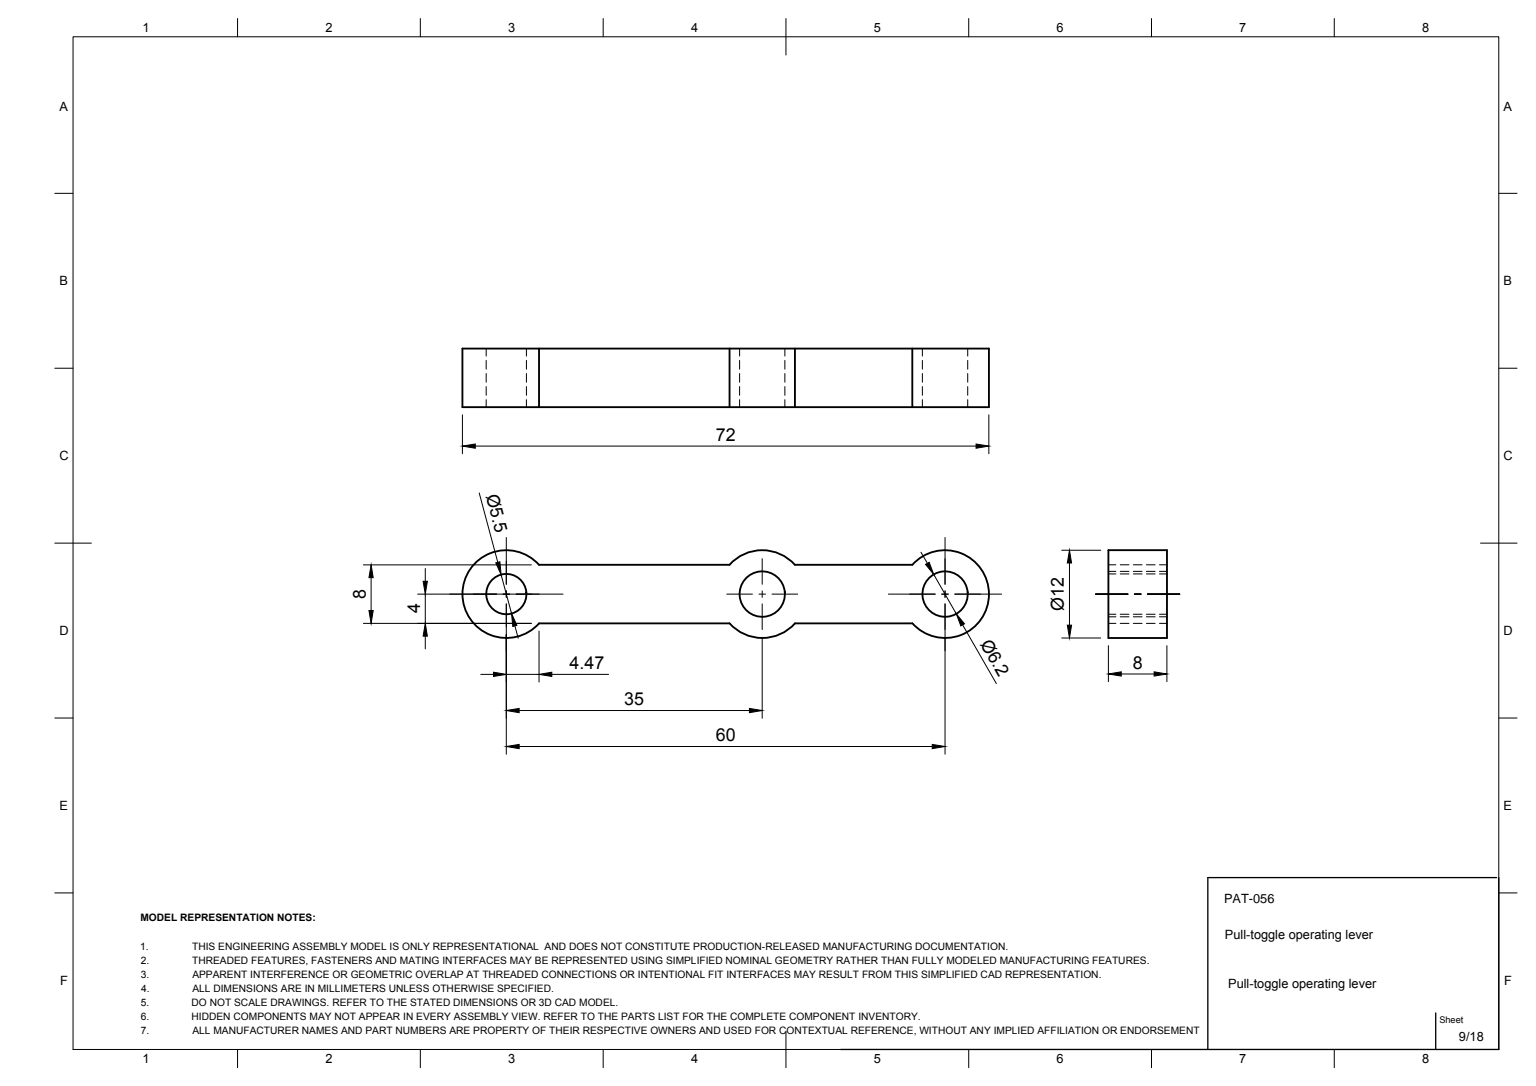
ISO-10303-21;
HEADER;
/* Generated by software containing ST-Developer
 * from STEP Tools, Inc. (www.steptools.com) 
 */

FILE_DESCRIPTION(
/* description */ ('Hook toggle clamp'),
/* implementation_level */ '2;1');

FILE_NAME(
/* name */ 'Pull-toggle operating lever.step',
/* time_stamp */ '2026-10-27T21:56:56-07:00',
/* author */ (''),
/* organization */ (''),
/* preprocessor_version */ 'ST-DEVELOPER v20.2',
/* originating_system */ 'Autodesk Translation Framework v15.17.0.0',
/* authorisation */ '');

FILE_SCHEMA (('AUTOMOTIVE_DESIGN { 1 0 10303 214 3 1 1 }'));
ENDSEC;

DATA;
#10=MECHANICAL_DESIGN_GEOMETRIC_PRESENTATION_REPRESENTATION('',(#192),#5458);
#158=SHAPE_REPRESENTATION_RELATIONSHIP('SRR','None',#5540,#175);
#175=ADVANCED_BREP_SHAPE_REPRESENTATION('',(#209),#5442);
#192=STYLED_ITEM('',(#5710),#209);
#209=MANIFOLD_SOLID_BREP('Body1',#2973);
#243=FACE_BOUND('',#653,.T.);
#244=FACE_BOUND('',#654,.T.);
#245=FACE_BOUND('',#655,.T.);
#246=FACE_BOUND('',#660,.T.);
#247=FACE_BOUND('',#661,.T.);
#248=FACE_BOUND('',#662,.T.);
#328=PLANE('',#3281);
#329=PLANE('',#3285);
#330=PLANE('',#3290);
#331=PLANE('',#3292);
#332=PLANE('',#3293);
#333=PLANE('',#3294);
#454=FACE_OUTER_BOUND('',#648,.T.);
#455=FACE_OUTER_BOUND('',#649,.T.);
#456=FACE_OUTER_BOUND('',#650,.T.);
#457=FACE_OUTER_BOUND('',#651,.T.);
#458=FACE_OUTER_BOUND('',#652,.T.);
#459=FACE_OUTER_BOUND('',#656,.T.);
#460=FACE_OUTER_BOUND('',#657,.T.);
#461=FACE_OUTER_BOUND('',#658,.T.);
#462=FACE_OUTER_BOUND('',#659,.T.);
#463=FACE_OUTER_BOUND('',#663,.T.);
#464=FACE_OUTER_BOUND('',#664,.T.);
#465=FACE_OUTER_BOUND('',#665,.T.);
#466=FACE_OUTER_BOUND('',#666,.T.);
#648=EDGE_LOOP('',(#2299,#2300,#2301,#2302));
#649=EDGE_LOOP('',(#2303,#2304,#2305,#2306));
#650=EDGE_LOOP('',(#2307,#2308,#2309,#2310));
#651=EDGE_LOOP('',(#2311,#2312,#2313,#2314));
#652=EDGE_LOOP('',(#2315,#2316,#2317,#2318,#2319,#2320,#2321,#2322));
#653=EDGE_LOOP('',(#2323));
#654=EDGE_LOOP('',(#2324));
#655=EDGE_LOOP('',(#2325));
#656=EDGE_LOOP('',(#2326,#2327,#2328,#2329));
#657=EDGE_LOOP('',(#2330,#2331,#2332,#2333));
#658=EDGE_LOOP('',(#2334,#2335,#2336,#2337));
#659=EDGE_LOOP('',(#2338,#2339,#2340,#2341,#2342,#2343,#2344,#2345));
#660=EDGE_LOOP('',(#2346));
#661=EDGE_LOOP('',(#2347));
#662=EDGE_LOOP('',(#2348));
#663=EDGE_LOOP('',(#2349,#2350,#2351,#2352));
#664=EDGE_LOOP('',(#2353,#2354,#2355,#2356));
#665=EDGE_LOOP('',(#2357,#2358,#2359,#2360));
#666=EDGE_LOOP('',(#2361,#2362,#2363,#2364));
#913=LINE('',#4750,#1150);
#914=LINE('',#4756,#1151);
#915=LINE('',#4762,#1152);
#916=LINE('',#4767,#1153);
#917=LINE('',#4771,#1154);
#918=LINE('',#4775,#1155);
#919=LINE('',#4779,#1156);
#920=LINE('',#4783,#1157);
#921=LINE('',#4786,#1158);
#922=LINE('',#4789,#1159);
#923=LINE('',#4790,#1160);
#924=LINE('',#4794,#1161);
#925=LINE('',#4797,#1162);
#926=LINE('',#4799,#1163);
#927=LINE('',#4802,#1164);
#928=LINE('',#4804,#1165);
#929=LINE('',#4807,#1166);
#930=LINE('',#4809,#1167);
#931=LINE('',#4811,#1168);
#1150=VECTOR('',#3819,0.275);
#1151=VECTOR('',#3826,0.31);
#1152=VECTOR('',#3833,0.31);
#1153=VECTOR('',#3838,1.);
#1154=VECTOR('',#3841,1.);
#1155=VECTOR('',#3846,1.);
#1156=VECTOR('',#3849,1.);
#1157=VECTOR('',#3852,1.);
#1158=VECTOR('',#3855,1.);
#1159=VECTOR('',#3858,1.);
#1160=VECTOR('',#3859,1.);
#1161=VECTOR('',#3864,1.);
#1162=VECTOR('',#3867,1.);
#1163=VECTOR('',#3868,1.);
#1164=VECTOR('',#3873,1.);
#1165=VECTOR('',#3874,1.);
#1166=VECTOR('',#3877,1.);
#1167=VECTOR('',#3880,1.);
#1168=VECTOR('',#3883,1.);
#1294=CIRCLE('',#3270,0.275);
#1295=CIRCLE('',#3271,0.275);
#1296=CIRCLE('',#3273,0.31);
#1297=CIRCLE('',#3274,0.31);
#1298=CIRCLE('',#3276,0.31);
#1299=CIRCLE('',#3277,0.31);
#1300=CIRCLE('',#3279,0.6);
#1301=CIRCLE('',#3280,0.6);
#1302=CIRCLE('',#3282,0.6);
#1303=CIRCLE('',#3283,0.6);
#1304=CIRCLE('',#3284,0.6);
#1305=CIRCLE('',#3287,0.6);
#1306=CIRCLE('',#3289,0.6);
#1307=CIRCLE('',#3291,0.6);
#1481=VERTEX_POINT('',#4747);
#1482=VERTEX_POINT('',#4749);
#1483=VERTEX_POINT('',#4753);
#1484=VERTEX_POINT('',#4755);
#1485=VERTEX_POINT('',#4759);
#1486=VERTEX_POINT('',#4761);
#1487=VERTEX_POINT('',#4765);
#1488=VERTEX_POINT('',#4766);
#1489=VERTEX_POINT('',#4768);
#1490=VERTEX_POINT('',#4770);
#1491=VERTEX_POINT('',#4774);
#1492=VERTEX_POINT('',#4776);
#1493=VERTEX_POINT('',#4778);
#1494=VERTEX_POINT('',#4780);
#1495=VERTEX_POINT('',#4782);
#1496=VERTEX_POINT('',#4784);
#1497=VERTEX_POINT('',#4788);
#1498=VERTEX_POINT('',#4792);
#1499=VERTEX_POINT('',#4796);
#1500=VERTEX_POINT('',#4798);
#1501=VERTEX_POINT('',#4803);
#1502=VERTEX_POINT('',#4805);
#1776=EDGE_CURVE('',#1481,#1481,#1294,.T.);
#1777=EDGE_CURVE('',#1481,#1482,#913,.T.);
#1778=EDGE_CURVE('',#1482,#1482,#1295,.T.);
#1779=EDGE_CURVE('',#1483,#1483,#1296,.T.);
#1780=EDGE_CURVE('',#1483,#1484,#914,.T.);
#1781=EDGE_CURVE('',#1484,#1484,#1297,.T.);
#1782=EDGE_CURVE('',#1485,#1485,#1298,.T.);
#1783=EDGE_CURVE('',#1485,#1486,#915,.T.);
#1784=EDGE_CURVE('',#1486,#1486,#1299,.T.);
#1785=EDGE_CURVE('',#1487,#1488,#916,.T.);
#1786=EDGE_CURVE('',#1489,#1487,#1300,.T.);
#1787=EDGE_CURVE('',#1490,#1489,#917,.T.);
#1788=EDGE_CURVE('',#1490,#1488,#1301,.T.);
#1789=EDGE_CURVE('',#1491,#1490,#918,.T.);
#1790=EDGE_CURVE('',#1492,#1491,#1302,.T.);
#1791=EDGE_CURVE('',#1493,#1492,#919,.T.);
#1792=EDGE_CURVE('',#1494,#1493,#1303,.T.);
#1793=EDGE_CURVE('',#1495,#1494,#920,.T.);
#1794=EDGE_CURVE('',#1496,#1495,#1304,.T.);
#1795=EDGE_CURVE('',#1488,#1496,#921,.T.);
#1796=EDGE_CURVE('',#1497,#1489,#922,.T.);
#1797=EDGE_CURVE('',#1497,#1491,#923,.T.);
#1798=EDGE_CURVE('',#1498,#1497,#1305,.T.);
#1799=EDGE_CURVE('',#1492,#1498,#924,.T.);
#1800=EDGE_CURVE('',#1496,#1499,#925,.T.);
#1801=EDGE_CURVE('',#1500,#1495,#926,.T.);
#1802=EDGE_CURVE('',#1499,#1500,#1306,.T.);
#1803=EDGE_CURVE('',#1487,#1499,#927,.T.);
#1804=EDGE_CURVE('',#1500,#1501,#928,.T.);
#1805=EDGE_CURVE('',#1501,#1502,#1307,.T.);
#1806=EDGE_CURVE('',#1502,#1498,#929,.T.);
#1807=EDGE_CURVE('',#1501,#1494,#930,.T.);
#1808=EDGE_CURVE('',#1493,#1502,#931,.T.);
#2299=ORIENTED_EDGE('',*,*,#1776,.F.);
#2300=ORIENTED_EDGE('',*,*,#1777,.T.);
#2301=ORIENTED_EDGE('',*,*,#1778,.F.);
#2302=ORIENTED_EDGE('',*,*,#1777,.F.);
#2303=ORIENTED_EDGE('',*,*,#1779,.F.);
#2304=ORIENTED_EDGE('',*,*,#1780,.T.);
#2305=ORIENTED_EDGE('',*,*,#1781,.F.);
#2306=ORIENTED_EDGE('',*,*,#1780,.F.);
#2307=ORIENTED_EDGE('',*,*,#1782,.F.);
#2308=ORIENTED_EDGE('',*,*,#1783,.T.);
#2309=ORIENTED_EDGE('',*,*,#1784,.F.);
#2310=ORIENTED_EDGE('',*,*,#1783,.F.);
#2311=ORIENTED_EDGE('',*,*,#1785,.F.);
#2312=ORIENTED_EDGE('',*,*,#1786,.F.);
#2313=ORIENTED_EDGE('',*,*,#1787,.F.);
#2314=ORIENTED_EDGE('',*,*,#1788,.T.);
#2315=ORIENTED_EDGE('',*,*,#1788,.F.);
#2316=ORIENTED_EDGE('',*,*,#1789,.F.);
#2317=ORIENTED_EDGE('',*,*,#1790,.F.);
#2318=ORIENTED_EDGE('',*,*,#1791,.F.);
#2319=ORIENTED_EDGE('',*,*,#1792,.F.);
#2320=ORIENTED_EDGE('',*,*,#1793,.F.);
#2321=ORIENTED_EDGE('',*,*,#1794,.F.);
#2322=ORIENTED_EDGE('',*,*,#1795,.F.);
#2323=ORIENTED_EDGE('',*,*,#1776,.T.);
#2324=ORIENTED_EDGE('',*,*,#1779,.T.);
#2325=ORIENTED_EDGE('',*,*,#1782,.T.);
#2326=ORIENTED_EDGE('',*,*,#1787,.T.);
#2327=ORIENTED_EDGE('',*,*,#1796,.F.);
#2328=ORIENTED_EDGE('',*,*,#1797,.T.);
#2329=ORIENTED_EDGE('',*,*,#1789,.T.);
#2330=ORIENTED_EDGE('',*,*,#1797,.F.);
#2331=ORIENTED_EDGE('',*,*,#1798,.F.);
#2332=ORIENTED_EDGE('',*,*,#1799,.F.);
#2333=ORIENTED_EDGE('',*,*,#1790,.T.);
#2334=ORIENTED_EDGE('',*,*,#1800,.F.);
#2335=ORIENTED_EDGE('',*,*,#1794,.T.);
#2336=ORIENTED_EDGE('',*,*,#1801,.F.);
#2337=ORIENTED_EDGE('',*,*,#1802,.F.);
#2338=ORIENTED_EDGE('',*,*,#1803,.T.);
#2339=ORIENTED_EDGE('',*,*,#1802,.T.);
#2340=ORIENTED_EDGE('',*,*,#1804,.T.);
#2341=ORIENTED_EDGE('',*,*,#1805,.T.);
#2342=ORIENTED_EDGE('',*,*,#1806,.T.);
#2343=ORIENTED_EDGE('',*,*,#1798,.T.);
#2344=ORIENTED_EDGE('',*,*,#1796,.T.);
#2345=ORIENTED_EDGE('',*,*,#1786,.T.);
#2346=ORIENTED_EDGE('',*,*,#1778,.T.);
#2347=ORIENTED_EDGE('',*,*,#1781,.T.);
#2348=ORIENTED_EDGE('',*,*,#1784,.T.);
#2349=ORIENTED_EDGE('',*,*,#1801,.T.);
#2350=ORIENTED_EDGE('',*,*,#1793,.T.);
#2351=ORIENTED_EDGE('',*,*,#1807,.F.);
#2352=ORIENTED_EDGE('',*,*,#1804,.F.);
#2353=ORIENTED_EDGE('',*,*,#1799,.T.);
#2354=ORIENTED_EDGE('',*,*,#1806,.F.);
#2355=ORIENTED_EDGE('',*,*,#1808,.F.);
#2356=ORIENTED_EDGE('',*,*,#1791,.T.);
#2357=ORIENTED_EDGE('',*,*,#1785,.T.);
#2358=ORIENTED_EDGE('',*,*,#1795,.T.);
#2359=ORIENTED_EDGE('',*,*,#1800,.T.);
#2360=ORIENTED_EDGE('',*,*,#1803,.F.);
#2361=ORIENTED_EDGE('',*,*,#1807,.T.);
#2362=ORIENTED_EDGE('',*,*,#1792,.T.);
#2363=ORIENTED_EDGE('',*,*,#1808,.T.);
#2364=ORIENTED_EDGE('',*,*,#1805,.F.);
#2759=CYLINDRICAL_SURFACE('',#3269,0.275);
#2760=CYLINDRICAL_SURFACE('',#3272,0.31);
#2761=CYLINDRICAL_SURFACE('',#3275,0.31);
#2762=CYLINDRICAL_SURFACE('',#3278,0.6);
#2763=CYLINDRICAL_SURFACE('',#3286,0.6);
#2764=CYLINDRICAL_SURFACE('',#3288,0.6);
#2765=CYLINDRICAL_SURFACE('',#3295,0.6);
#2858=ADVANCED_FACE('',(#454),#2759,.F.);
#2859=ADVANCED_FACE('',(#455),#2760,.F.);
#2860=ADVANCED_FACE('',(#456),#2761,.F.);
#2861=ADVANCED_FACE('',(#457),#2762,.T.);
#2862=ADVANCED_FACE('',(#458,#243,#244,#245),#328,.F.);
#2863=ADVANCED_FACE('',(#459),#329,.T.);
#2864=ADVANCED_FACE('',(#460),#2763,.T.);
#2865=ADVANCED_FACE('',(#461),#2764,.T.);
#2866=ADVANCED_FACE('',(#462,#246,#247,#248),#330,.T.);
#2867=ADVANCED_FACE('',(#463),#331,.T.);
#2868=ADVANCED_FACE('',(#464),#332,.T.);
#2869=ADVANCED_FACE('',(#465),#333,.T.);
#2870=ADVANCED_FACE('',(#466),#2765,.T.);
#2973=CLOSED_SHELL('',(#2858,#2859,#2860,#2861,#2862,#2863,#2864,#2865,
#2866,#2867,#2868,#2869,#2870));
#3268=AXIS2_PLACEMENT_3D('',#4745,#3813,#3814);
#3269=AXIS2_PLACEMENT_3D('',#4746,#3815,#3816);
#3270=AXIS2_PLACEMENT_3D('',#4748,#3817,#3818);
#3271=AXIS2_PLACEMENT_3D('',#4751,#3820,#3821);
#3272=AXIS2_PLACEMENT_3D('',#4752,#3822,#3823);
#3273=AXIS2_PLACEMENT_3D('',#4754,#3824,#3825);
#3274=AXIS2_PLACEMENT_3D('',#4757,#3827,#3828);
#3275=AXIS2_PLACEMENT_3D('',#4758,#3829,#3830);
#3276=AXIS2_PLACEMENT_3D('',#4760,#3831,#3832);
#3277=AXIS2_PLACEMENT_3D('',#4763,#3834,#3835);
#3278=AXIS2_PLACEMENT_3D('',#4764,#3836,#3837);
#3279=AXIS2_PLACEMENT_3D('',#4769,#3839,#3840);
#3280=AXIS2_PLACEMENT_3D('',#4772,#3842,#3843);
#3281=AXIS2_PLACEMENT_3D('',#4773,#3844,#3845);
#3282=AXIS2_PLACEMENT_3D('',#4777,#3847,#3848);
#3283=AXIS2_PLACEMENT_3D('',#4781,#3850,#3851);
#3284=AXIS2_PLACEMENT_3D('',#4785,#3853,#3854);
#3285=AXIS2_PLACEMENT_3D('',#4787,#3856,#3857);
#3286=AXIS2_PLACEMENT_3D('',#4791,#3860,#3861);
#3287=AXIS2_PLACEMENT_3D('',#4793,#3862,#3863);
#3288=AXIS2_PLACEMENT_3D('',#4795,#3865,#3866);
#3289=AXIS2_PLACEMENT_3D('',#4800,#3869,#3870);
#3290=AXIS2_PLACEMENT_3D('',#4801,#3871,#3872);
#3291=AXIS2_PLACEMENT_3D('',#4806,#3875,#3876);
#3292=AXIS2_PLACEMENT_3D('',#4808,#3878,#3879);
#3293=AXIS2_PLACEMENT_3D('',#4810,#3881,#3882);
#3294=AXIS2_PLACEMENT_3D('',#4812,#3884,#3885);
#3295=AXIS2_PLACEMENT_3D('',#4813,#3886,#3887);
#3813=DIRECTION('axis',(0.,0.,1.));
#3814=DIRECTION('refdir',(1.,0.,0.));
#3815=DIRECTION('center_axis',(0.,1.,0.));
#3816=DIRECTION('ref_axis',(1.,0.,0.));
#3817=DIRECTION('center_axis',(0.,1.,0.));
#3818=DIRECTION('ref_axis',(1.,0.,0.));
#3819=DIRECTION('',(0.,1.,0.));
#3820=DIRECTION('center_axis',(0.,-1.,0.));
#3821=DIRECTION('ref_axis',(1.,0.,0.));
#3822=DIRECTION('center_axis',(0.,1.,0.));
#3823=DIRECTION('ref_axis',(1.,0.,0.));
#3824=DIRECTION('center_axis',(0.,1.,0.));
#3825=DIRECTION('ref_axis',(1.,0.,0.));
#3826=DIRECTION('',(0.,1.,0.));
#3827=DIRECTION('center_axis',(0.,-1.,0.));
#3828=DIRECTION('ref_axis',(1.,0.,0.));
#3829=DIRECTION('center_axis',(0.,1.,0.));
#3830=DIRECTION('ref_axis',(1.,0.,0.));
#3831=DIRECTION('center_axis',(0.,1.,0.));
#3832=DIRECTION('ref_axis',(1.,0.,0.));
#3833=DIRECTION('',(0.,1.,0.));
#3834=DIRECTION('center_axis',(0.,-1.,0.));
#3835=DIRECTION('ref_axis',(1.,0.,0.));
#3836=DIRECTION('center_axis',(0.,1.,0.));
#3837=DIRECTION('ref_axis',(-0.996194698091745,0.,-0.0871557427476579));
#3838=DIRECTION('',(0.,-1.,0.));
#3839=DIRECTION('center_axis',(0.,1.,0.));
#3840=DIRECTION('ref_axis',(1.,0.,0.));
#3841=DIRECTION('',(0.,1.,0.));
#3842=DIRECTION('center_axis',(0.,1.,0.));
#3843=DIRECTION('ref_axis',(1.,0.,0.));
#3844=DIRECTION('center_axis',(0.,1.,0.));
#3845=DIRECTION('ref_axis',(1.,0.,0.));
#3846=DIRECTION('',(-0.996194698091746,0.,-0.0871557427476579));
#3847=DIRECTION('center_axis',(0.,1.,0.));
#3848=DIRECTION('ref_axis',(1.,0.,0.));
#3849=DIRECTION('',(-0.996194698091746,0.,-0.0871557427476579));
#3850=DIRECTION('center_axis',(0.,1.,0.));
#3851=DIRECTION('ref_axis',(1.,0.,0.));
#3852=DIRECTION('',(0.996194698091746,0.,0.087155742747658));
#3853=DIRECTION('center_axis',(0.,1.,0.));
#3854=DIRECTION('ref_axis',(1.,0.,0.));
#3855=DIRECTION('',(0.996194698091746,0.,0.087155742747658));
#3856=DIRECTION('center_axis',(0.0871557427476579,0.,-0.996194698091746));
#3857=DIRECTION('ref_axis',(-0.996194698091746,0.,-0.0871557427476579));
#3858=DIRECTION('',(-0.996194698091746,0.,-0.0871557427476579));
#3859=DIRECTION('',(0.,-1.,0.));
#3860=DIRECTION('center_axis',(0.,1.,0.));
#3861=DIRECTION('ref_axis',(1.,0.,0.));
#3862=DIRECTION('center_axis',(0.,1.,0.));
#3863=DIRECTION('ref_axis',(1.,0.,0.));
#3864=DIRECTION('',(0.,1.,0.));
#3865=DIRECTION('center_axis',(0.,1.,0.));
#3866=DIRECTION('ref_axis',(1.,0.,0.));
#3867=DIRECTION('',(0.,1.,0.));
#3868=DIRECTION('',(0.,-1.,0.));
#3869=DIRECTION('center_axis',(0.,1.,0.));
#3870=DIRECTION('ref_axis',(1.,0.,0.));
#3871=DIRECTION('center_axis',(0.,1.,0.));
#3872=DIRECTION('ref_axis',(1.,0.,0.));
#3873=DIRECTION('',(0.996194698091746,0.,0.087155742747658));
#3874=DIRECTION('',(0.996194698091746,0.,0.087155742747658));
#3875=DIRECTION('center_axis',(0.,1.,0.));
#3876=DIRECTION('ref_axis',(1.,0.,0.));
#3877=DIRECTION('',(-0.996194698091746,0.,-0.0871557427476579));
#3878=DIRECTION('center_axis',(-0.087155742747658,0.,0.996194698091746));
#3879=DIRECTION('ref_axis',(0.996194698091746,0.,0.087155742747658));
#3880=DIRECTION('',(0.,-1.,0.));
#3881=DIRECTION('center_axis',(0.0871557427476579,0.,-0.996194698091746));
#3882=DIRECTION('ref_axis',(-0.996194698091746,0.,-0.0871557427476579));
#3883=DIRECTION('',(0.,1.,0.));
#3884=DIRECTION('center_axis',(-0.087155742747658,0.,0.996194698091746));
#3885=DIRECTION('ref_axis',(0.996194698091746,0.,0.087155742747658));
#3886=DIRECTION('center_axis',(0.,1.,0.));
#3887=DIRECTION('ref_axis',(1.,0.,0.));
#4745=CARTESIAN_POINT('',(0.,0.,0.));
#4746=CARTESIAN_POINT('Origin',(-5.97716818855047,-0.5,1.97706554351405));
#4747=CARTESIAN_POINT('',(-6.25216818855047,-0.4,1.97706554351405));
#4748=CARTESIAN_POINT('Origin',(-5.97716818855047,-0.4,1.97706554351405));
#4749=CARTESIAN_POINT('',(-6.25216818855047,0.4,1.97706554351405));
#4750=CARTESIAN_POINT('',(-6.25216818855047,-0.5,1.97706554351405));
#4751=CARTESIAN_POINT('Origin',(-5.97716818855047,0.4,1.97706554351405));
#4752=CARTESIAN_POINT('Origin',(0.,-0.5,2.5));
#4753=CARTESIAN_POINT('',(-0.31,-0.4,2.5));
#4754=CARTESIAN_POINT('Origin',(0.,-0.4,2.5));
#4755=CARTESIAN_POINT('',(-0.31,0.4,2.5));
#4756=CARTESIAN_POINT('',(-0.31,-0.5,2.5));
#4757=CARTESIAN_POINT('Origin',(0.,0.4,2.5));
#4758=CARTESIAN_POINT('Origin',(-2.49048674522936,-0.5,2.28211064313086));
#4759=CARTESIAN_POINT('',(-2.80048674522936,-0.4,2.28211064313086));
#4760=CARTESIAN_POINT('Origin',(-2.49048674522936,-0.4,2.28211064313086));
#4761=CARTESIAN_POINT('',(-2.80048674522936,0.4,2.28211064313086));
#4762=CARTESIAN_POINT('',(-2.80048674522936,-0.5,2.28211064313086));
#4763=CARTESIAN_POINT('Origin',(-2.49048674522936,0.4,2.28211064313086));
#4764=CARTESIAN_POINT('Origin',(-5.97716818855047,-0.4,1.97706554351405));
#4765=CARTESIAN_POINT('',(-5.56651867289793,0.4,2.4145206558334));
#4766=CARTESIAN_POINT('',(-5.56651867289793,-0.4,2.4145206558334));
#4767=CARTESIAN_POINT('',(-5.56651867289793,-0.4,2.4145206558334));
#4768=CARTESIAN_POINT('',(-5.49679407869981,0.4,1.61756489736));
#4769=CARTESIAN_POINT('Origin',(-5.97716818855047,0.4,1.97706554351405));
#4770=CARTESIAN_POINT('',(-5.49679407869981,-0.4,1.61756489736));
#4771=CARTESIAN_POINT('',(-5.49679407869981,-0.4,1.61756489736));
#4772=CARTESIAN_POINT('Origin',(-5.97716818855047,-0.4,1.97706554351405));
#4773=CARTESIAN_POINT('Origin',(0.,-0.4,2.5));
#4774=CARTESIAN_POINT('',(-2.90113626088191,-0.4,1.84465553081151));
#4775=CARTESIAN_POINT('',(0.0348622970990632,-0.4,2.1015221207633));
#4776=CARTESIAN_POINT('',(-2.0101126353787,-0.4,1.92260999697681));
#4777=CARTESIAN_POINT('Origin',(-2.49048674522936,-0.4,2.28211064313086));
#4778=CARTESIAN_POINT('',(-0.410649515652541,-0.4,2.06254488768065));
#4779=CARTESIAN_POINT('',(0.0348622970990632,-0.4,2.1015221207633));
#4780=CARTESIAN_POINT('',(-0.480374109850668,-0.4,2.85950064615405));
#4781=CARTESIAN_POINT('Origin',(0.,-0.4,2.5));
#4782=CARTESIAN_POINT('',(-2.07983722957682,-0.4,2.7195657554502));
#4783=CARTESIAN_POINT('',(-6.01203048564954,-0.4,2.37554342275075));
#4784=CARTESIAN_POINT('',(-2.97086085508003,-0.4,2.6416112892849));
#4785=CARTESIAN_POINT('Origin',(-2.49048674522936,-0.4,2.28211064313086));
#4786=CARTESIAN_POINT('',(-6.01203048564954,-0.4,2.37554342275075));
#4787=CARTESIAN_POINT('Origin',(0.0348622970990632,-0.4,2.1015221207633));
#4788=CARTESIAN_POINT('',(-2.90113626088191,0.4,1.84465553081151));
#4789=CARTESIAN_POINT('',(0.0348622970990632,0.4,2.1015221207633));
#4790=CARTESIAN_POINT('',(-2.90113626088191,-0.4,1.84465553081151));
#4791=CARTESIAN_POINT('Origin',(-2.49048674522936,-0.4,2.28211064313086));
#4792=CARTESIAN_POINT('',(-2.0101126353787,0.4,1.92260999697681));
#4793=CARTESIAN_POINT('Origin',(-2.49048674522936,0.4,2.28211064313086));
#4794=CARTESIAN_POINT('',(-2.0101126353787,-0.4,1.92260999697681));
#4795=CARTESIAN_POINT('Origin',(-2.49048674522936,-0.4,2.28211064313086));
#4796=CARTESIAN_POINT('',(-2.97086085508003,0.4,2.6416112892849));
#4797=CARTESIAN_POINT('',(-2.97086085508003,-0.4,2.6416112892849));
#4798=CARTESIAN_POINT('',(-2.07983722957682,0.4,2.7195657554502));
#4799=CARTESIAN_POINT('',(-2.07983722957682,-0.4,2.7195657554502));
#4800=CARTESIAN_POINT('Origin',(-2.49048674522936,0.4,2.28211064313086));
#4801=CARTESIAN_POINT('Origin',(0.,0.4,2.5));
#4802=CARTESIAN_POINT('',(-6.01203048564954,0.4,2.37554342275075));
#4803=CARTESIAN_POINT('',(-0.480374109850668,0.4,2.85950064615405));
#4804=CARTESIAN_POINT('',(-6.01203048564954,0.4,2.37554342275075));
#4805=CARTESIAN_POINT('',(-0.410649515652541,0.4,2.06254488768065));
#4806=CARTESIAN_POINT('Origin',(0.,0.4,2.5));
#4807=CARTESIAN_POINT('',(0.0348622970990632,0.4,2.1015221207633));
#4808=CARTESIAN_POINT('Origin',(-6.01203048564954,-0.4,2.37554342275075));
#4809=CARTESIAN_POINT('',(-0.480374109850667,-0.4,2.85950064615405));
#4810=CARTESIAN_POINT('Origin',(0.0348622970990632,-0.4,2.1015221207633));
#4811=CARTESIAN_POINT('',(-0.410649515652541,-0.4,2.06254488768065));
#4812=CARTESIAN_POINT('Origin',(-6.01203048564954,-0.4,2.37554342275075));
#4813=CARTESIAN_POINT('Origin',(0.,-0.4,2.5));
#5419=UNCERTAINTY_MEASURE_WITH_UNIT(LENGTH_MEASURE(0.001),#5459,
'DISTANCE_ACCURACY_VALUE',
'Maximum model space distance between geometric entities at asserted c
onnectivities');
#5435=UNCERTAINTY_MEASURE_WITH_UNIT(LENGTH_MEASURE(0.001),#5459,
'DISTANCE_ACCURACY_VALUE',
'Maximum model space distance between geometric entities at asserted c
onnectivities');
#5442=(
GEOMETRIC_REPRESENTATION_CONTEXT(3)
GLOBAL_UNCERTAINTY_ASSIGNED_CONTEXT((#5419))
GLOBAL_UNIT_ASSIGNED_CONTEXT((#5459,#5461,#5462))
REPRESENTATION_CONTEXT('','3D')
);
#5458=(
GEOMETRIC_REPRESENTATION_CONTEXT(3)
GLOBAL_UNCERTAINTY_ASSIGNED_CONTEXT((#5435))
GLOBAL_UNIT_ASSIGNED_CONTEXT((#5459,#5461,#5462))
REPRESENTATION_CONTEXT('','3D')
);
#5459=(
LENGTH_UNIT()
NAMED_UNIT(*)
SI_UNIT(.CENTI.,.METRE.)
);
#5461=(
NAMED_UNIT(*)
PLANE_ANGLE_UNIT()
SI_UNIT($,.RADIAN.)
);
#5462=(
NAMED_UNIT(*)
SI_UNIT($,.STERADIAN.)
SOLID_ANGLE_UNIT()
);
#5469=SHAPE_DEFINITION_REPRESENTATION(#5491,#5540);
#5491=PRODUCT_DEFINITION_SHAPE('',$,#5563);
#5540=SHAPE_REPRESENTATION('',(#3268),#5442);
#5556=PRODUCT_DEFINITION_CONTEXT('part definition',#5624,'design');
#5563=PRODUCT_DEFINITION('Pull-toggle operating lever',
'Pull-toggle operating lever',#5585,#5556);
#5585=PRODUCT_DEFINITION_FORMATION('',$,#5632);
#5624=APPLICATION_CONTEXT(
'Core Data for Automotive Mechanical Design Process');
#5625=PRODUCT_CONTEXT('part definition',#5624,'mechanical');
#5632=PRODUCT('Pull-toggle operating lever',
'Pull-toggle operating lever','Pull-toggle operating lever',(#5625));
#5704=COLOUR_RGB('Sky Blue',0.24,0.69,0.87);
#5705=FILL_AREA_STYLE_COLOUR('',#5704);
#5706=FILL_AREA_STYLE('',(#5705));
#5707=SURFACE_STYLE_FILL_AREA(#5706);
#5708=SURFACE_SIDE_STYLE('',(#5707));
#5709=SURFACE_STYLE_USAGE(.BOTH.,#5708);
#5710=PRESENTATION_STYLE_ASSIGNMENT((#5709));
ENDSEC;
END-ISO-10303-21;
